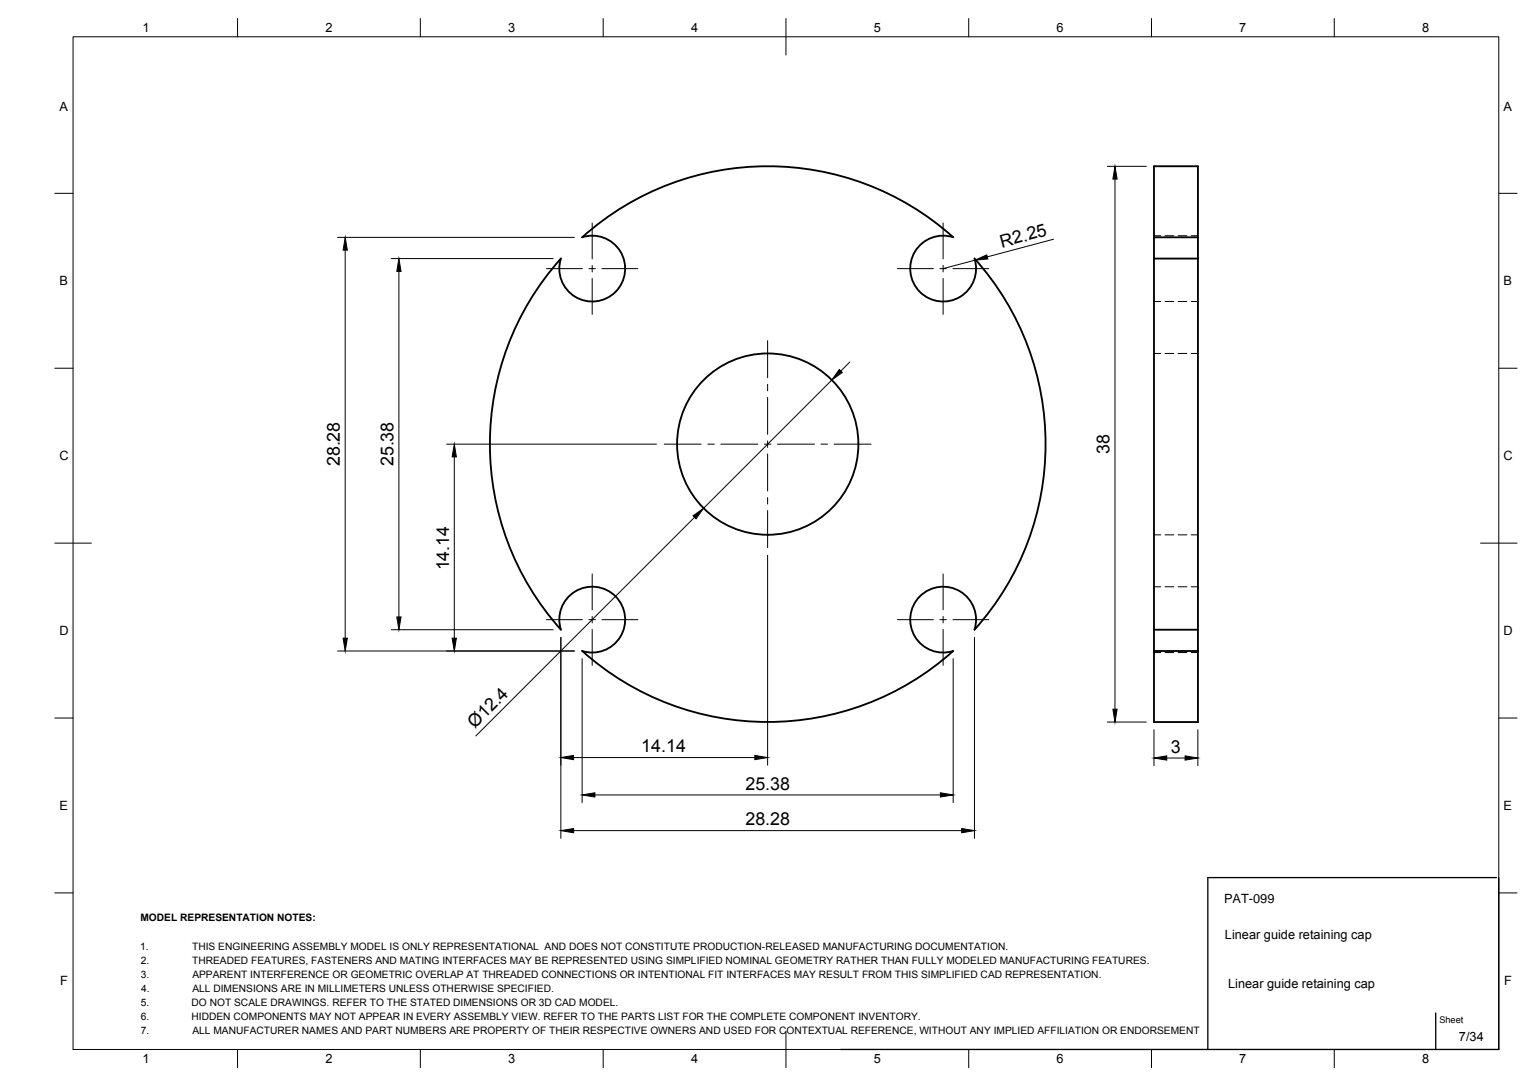
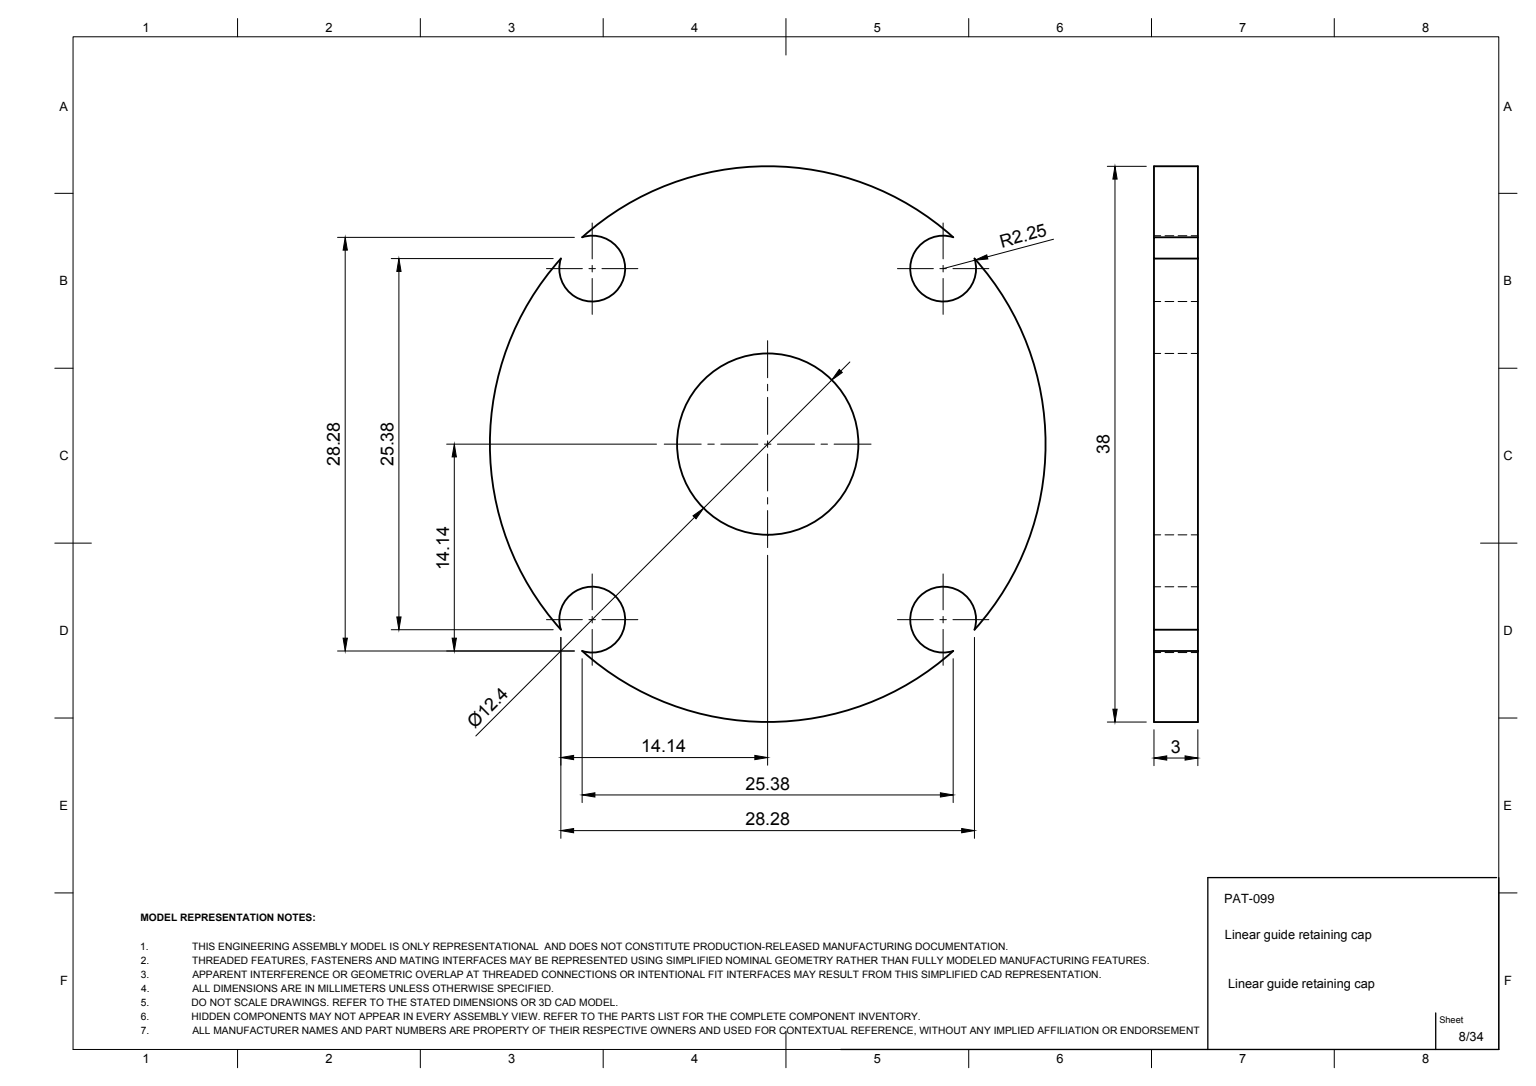
ISO-10303-21;
HEADER;
/* Generated by software containing ST-Developer
 * from STEP Tools, Inc. (www.steptools.com) 
 */

FILE_DESCRIPTION(
/* description */ ('PAT-099'),
/* implementation_level */ '2;1');

FILE_NAME(
/* name */ 'Linear guide retaining cap.step',
/* time_stamp */ '2026-10-29T17:25:42-07:00',
/* author */ (''),
/* organization */ (''),
/* preprocessor_version */ 'ST-DEVELOPER v20.2',
/* originating_system */ 'Autodesk Translation Framework v15.17.0.0',
/* authorisation */ '');

FILE_SCHEMA (('AUTOMOTIVE_DESIGN { 1 0 10303 214 3 1 1 }'));
ENDSEC;

DATA;
#10=MECHANICAL_DESIGN_GEOMETRIC_PRESENTATION_REPRESENTATION('',(#339),#11035);
#289=SHAPE_REPRESENTATION_RELATIONSHIP('SRR','None',#11157,#314);
#314=ADVANCED_BREP_SHAPE_REPRESENTATION('',(#372),#11007);
#339=STYLED_ITEM('',(#11379),#372);
#372=MANIFOLD_SOLID_BREP('Body1',#4707);
#441=FACE_BOUND('',#1018,.T.);
#442=FACE_BOUND('',#1025,.T.);
#537=PLANE('',#5096);
#538=PLANE('',#5112);
#692=FACE_OUTER_BOUND('',#1013,.T.);
#693=FACE_OUTER_BOUND('',#1014,.T.);
#694=FACE_OUTER_BOUND('',#1015,.T.);
#695=FACE_OUTER_BOUND('',#1016,.T.);
#696=FACE_OUTER_BOUND('',#1017,.T.);
#697=FACE_OUTER_BOUND('',#1019,.T.);
#698=FACE_OUTER_BOUND('',#1020,.T.);
#699=FACE_OUTER_BOUND('',#1021,.T.);
#700=FACE_OUTER_BOUND('',#1022,.T.);
#701=FACE_OUTER_BOUND('',#1023,.T.);
#702=FACE_OUTER_BOUND('',#1024,.T.);
#1013=EDGE_LOOP('',(#3313,#3314,#3315,#3316));
#1014=EDGE_LOOP('',(#3317,#3318,#3319,#3320));
#1015=EDGE_LOOP('',(#3321,#3322,#3323,#3324));
#1016=EDGE_LOOP('',(#3325,#3326,#3327,#3328));
#1017=EDGE_LOOP('',(#3329,#3330,#3331,#3332,#3333,#3334,#3335,#3336));
#1018=EDGE_LOOP('',(#3337));
#1019=EDGE_LOOP('',(#3338,#3339,#3340,#3341));
#1020=EDGE_LOOP('',(#3342,#3343,#3344,#3345));
#1021=EDGE_LOOP('',(#3346,#3347,#3348,#3349));
#1022=EDGE_LOOP('',(#3350,#3351,#3352,#3353));
#1023=EDGE_LOOP('',(#3354,#3355,#3356,#3357));
#1024=EDGE_LOOP('',(#3358,#3359,#3360,#3361,#3362,#3363,#3364,#3365));
#1025=EDGE_LOOP('',(#3366));
#1386=LINE('',#7806,#1638);
#1387=LINE('',#7810,#1639);
#1388=LINE('',#7815,#1640);
#1389=LINE('',#7819,#1641);
#1390=LINE('',#7824,#1642);
#1391=LINE('',#7828,#1643);
#1392=LINE('',#7833,#1644);
#1393=LINE('',#7837,#1645);
#1394=LINE('',#7857,#1646);
#1638=VECTOR('',#5849,1.);
#1639=VECTOR('',#5852,1.);
#1640=VECTOR('',#5857,1.);
#1641=VECTOR('',#5860,1.);
#1642=VECTOR('',#5865,1.);
#1643=VECTOR('',#5868,1.);
#1644=VECTOR('',#5873,1.);
#1645=VECTOR('',#5876,1.);
#1646=VECTOR('',#5911,0.62);
#1877=CIRCLE('',#5085,0.225);
#1878=CIRCLE('',#5086,0.225);
#1879=CIRCLE('',#5088,0.225);
#1880=CIRCLE('',#5089,0.225);
#1881=CIRCLE('',#5091,0.225);
#1882=CIRCLE('',#5092,0.225);
#1883=CIRCLE('',#5094,0.225);
#1884=CIRCLE('',#5095,0.225);
#1885=CIRCLE('',#5097,1.9);
#1886=CIRCLE('',#5098,1.9);
#1887=CIRCLE('',#5099,1.9);
#1888=CIRCLE('',#5100,1.9);
#1889=CIRCLE('',#5101,0.62);
#1890=CIRCLE('',#5103,1.9);
#1891=CIRCLE('',#5105,1.9);
#1892=CIRCLE('',#5107,1.9);
#1893=CIRCLE('',#5109,1.9);
#1894=CIRCLE('',#5111,0.62);
#2202=VERTEX_POINT('',#7804);
#2203=VERTEX_POINT('',#7805);
#2204=VERTEX_POINT('',#7807);
#2205=VERTEX_POINT('',#7809);
#2206=VERTEX_POINT('',#7813);
#2207=VERTEX_POINT('',#7814);
#2208=VERTEX_POINT('',#7816);
#2209=VERTEX_POINT('',#7818);
#2210=VERTEX_POINT('',#7822);
#2211=VERTEX_POINT('',#7823);
#2212=VERTEX_POINT('',#7825);
#2213=VERTEX_POINT('',#7827);
#2214=VERTEX_POINT('',#7831);
#2215=VERTEX_POINT('',#7832);
#2216=VERTEX_POINT('',#7834);
#2217=VERTEX_POINT('',#7836);
#2218=VERTEX_POINT('',#7844);
#2219=VERTEX_POINT('',#7855);
#2633=EDGE_CURVE('',#2202,#2203,#1386,.T.);
#2634=EDGE_CURVE('',#2204,#2202,#1877,.T.);
#2635=EDGE_CURVE('',#2205,#2204,#1387,.T.);
#2636=EDGE_CURVE('',#2203,#2205,#1878,.T.);
#2637=EDGE_CURVE('',#2206,#2207,#1388,.T.);
#2638=EDGE_CURVE('',#2208,#2206,#1879,.T.);
#2639=EDGE_CURVE('',#2209,#2208,#1389,.T.);
#2640=EDGE_CURVE('',#2207,#2209,#1880,.T.);
#2641=EDGE_CURVE('',#2210,#2211,#1390,.T.);
#2642=EDGE_CURVE('',#2212,#2210,#1881,.T.);
#2643=EDGE_CURVE('',#2213,#2212,#1391,.T.);
#2644=EDGE_CURVE('',#2211,#2213,#1882,.T.);
#2645=EDGE_CURVE('',#2214,#2215,#1392,.T.);
#2646=EDGE_CURVE('',#2216,#2214,#1883,.T.);
#2647=EDGE_CURVE('',#2217,#2216,#1393,.T.);
#2648=EDGE_CURVE('',#2215,#2217,#1884,.T.);
#2649=EDGE_CURVE('',#2212,#2202,#1885,.T.);
#2650=EDGE_CURVE('',#2208,#2210,#1886,.T.);
#2651=EDGE_CURVE('',#2216,#2206,#1887,.T.);
#2652=EDGE_CURVE('',#2204,#2214,#1888,.T.);
#2653=EDGE_CURVE('',#2218,#2218,#1889,.T.);
#2654=EDGE_CURVE('',#2217,#2207,#1890,.T.);
#2655=EDGE_CURVE('',#2209,#2211,#1891,.T.);
#2656=EDGE_CURVE('',#2213,#2203,#1892,.T.);
#2657=EDGE_CURVE('',#2205,#2215,#1893,.T.);
#2658=EDGE_CURVE('',#2219,#2219,#1894,.T.);
#2659=EDGE_CURVE('',#2219,#2218,#1394,.T.);
#3313=ORIENTED_EDGE('',*,*,#2633,.F.);
#3314=ORIENTED_EDGE('',*,*,#2634,.F.);
#3315=ORIENTED_EDGE('',*,*,#2635,.F.);
#3316=ORIENTED_EDGE('',*,*,#2636,.F.);
#3317=ORIENTED_EDGE('',*,*,#2637,.F.);
#3318=ORIENTED_EDGE('',*,*,#2638,.F.);
#3319=ORIENTED_EDGE('',*,*,#2639,.F.);
#3320=ORIENTED_EDGE('',*,*,#2640,.F.);
#3321=ORIENTED_EDGE('',*,*,#2641,.F.);
#3322=ORIENTED_EDGE('',*,*,#2642,.F.);
#3323=ORIENTED_EDGE('',*,*,#2643,.F.);
#3324=ORIENTED_EDGE('',*,*,#2644,.F.);
#3325=ORIENTED_EDGE('',*,*,#2645,.F.);
#3326=ORIENTED_EDGE('',*,*,#2646,.F.);
#3327=ORIENTED_EDGE('',*,*,#2647,.F.);
#3328=ORIENTED_EDGE('',*,*,#2648,.F.);
#3329=ORIENTED_EDGE('',*,*,#2634,.T.);
#3330=ORIENTED_EDGE('',*,*,#2649,.F.);
#3331=ORIENTED_EDGE('',*,*,#2642,.T.);
#3332=ORIENTED_EDGE('',*,*,#2650,.F.);
#3333=ORIENTED_EDGE('',*,*,#2638,.T.);
#3334=ORIENTED_EDGE('',*,*,#2651,.F.);
#3335=ORIENTED_EDGE('',*,*,#2646,.T.);
#3336=ORIENTED_EDGE('',*,*,#2652,.F.);
#3337=ORIENTED_EDGE('',*,*,#2653,.F.);
#3338=ORIENTED_EDGE('',*,*,#2637,.T.);
#3339=ORIENTED_EDGE('',*,*,#2654,.F.);
#3340=ORIENTED_EDGE('',*,*,#2647,.T.);
#3341=ORIENTED_EDGE('',*,*,#2651,.T.);
#3342=ORIENTED_EDGE('',*,*,#2639,.T.);
#3343=ORIENTED_EDGE('',*,*,#2650,.T.);
#3344=ORIENTED_EDGE('',*,*,#2641,.T.);
#3345=ORIENTED_EDGE('',*,*,#2655,.F.);
#3346=ORIENTED_EDGE('',*,*,#2633,.T.);
#3347=ORIENTED_EDGE('',*,*,#2656,.F.);
#3348=ORIENTED_EDGE('',*,*,#2643,.T.);
#3349=ORIENTED_EDGE('',*,*,#2649,.T.);
#3350=ORIENTED_EDGE('',*,*,#2635,.T.);
#3351=ORIENTED_EDGE('',*,*,#2652,.T.);
#3352=ORIENTED_EDGE('',*,*,#2645,.T.);
#3353=ORIENTED_EDGE('',*,*,#2657,.F.);
#3354=ORIENTED_EDGE('',*,*,#2658,.F.);
#3355=ORIENTED_EDGE('',*,*,#2659,.T.);
#3356=ORIENTED_EDGE('',*,*,#2653,.T.);
#3357=ORIENTED_EDGE('',*,*,#2659,.F.);
#3358=ORIENTED_EDGE('',*,*,#2636,.T.);
#3359=ORIENTED_EDGE('',*,*,#2657,.T.);
#3360=ORIENTED_EDGE('',*,*,#2648,.T.);
#3361=ORIENTED_EDGE('',*,*,#2654,.T.);
#3362=ORIENTED_EDGE('',*,*,#2640,.T.);
#3363=ORIENTED_EDGE('',*,*,#2655,.T.);
#3364=ORIENTED_EDGE('',*,*,#2644,.T.);
#3365=ORIENTED_EDGE('',*,*,#2656,.T.);
#3366=ORIENTED_EDGE('',*,*,#2658,.T.);
#4328=CYLINDRICAL_SURFACE('',#5084,0.225);
#4329=CYLINDRICAL_SURFACE('',#5087,0.225);
#4330=CYLINDRICAL_SURFACE('',#5090,0.225);
#4331=CYLINDRICAL_SURFACE('',#5093,0.225);
#4332=CYLINDRICAL_SURFACE('',#5102,1.9);
#4333=CYLINDRICAL_SURFACE('',#5104,1.9);
#4334=CYLINDRICAL_SURFACE('',#5106,1.9);
#4335=CYLINDRICAL_SURFACE('',#5108,1.9);
#4336=CYLINDRICAL_SURFACE('',#5110,0.62);
#4457=ADVANCED_FACE('',(#692),#4328,.F.);
#4458=ADVANCED_FACE('',(#693),#4329,.F.);
#4459=ADVANCED_FACE('',(#694),#4330,.F.);
#4460=ADVANCED_FACE('',(#695),#4331,.F.);
#4461=ADVANCED_FACE('',(#696,#441),#537,.F.);
#4462=ADVANCED_FACE('',(#697),#4332,.T.);
#4463=ADVANCED_FACE('',(#698),#4333,.T.);
#4464=ADVANCED_FACE('',(#699),#4334,.T.);
#4465=ADVANCED_FACE('',(#700),#4335,.T.);
#4466=ADVANCED_FACE('',(#701),#4336,.F.);
#4467=ADVANCED_FACE('',(#702,#442),#538,.T.);
#4707=CLOSED_SHELL('',(#4457,#4458,#4459,#4460,#4461,#4462,#4463,#4464,
#4465,#4466,#4467));
#5083=AXIS2_PLACEMENT_3D('',#7802,#5845,#5846);
#5084=AXIS2_PLACEMENT_3D('',#7803,#5847,#5848);
#5085=AXIS2_PLACEMENT_3D('',#7808,#5850,#5851);
#5086=AXIS2_PLACEMENT_3D('',#7811,#5853,#5854);
#5087=AXIS2_PLACEMENT_3D('',#7812,#5855,#5856);
#5088=AXIS2_PLACEMENT_3D('',#7817,#5858,#5859);
#5089=AXIS2_PLACEMENT_3D('',#7820,#5861,#5862);
#5090=AXIS2_PLACEMENT_3D('',#7821,#5863,#5864);
#5091=AXIS2_PLACEMENT_3D('',#7826,#5866,#5867);
#5092=AXIS2_PLACEMENT_3D('',#7829,#5869,#5870);
#5093=AXIS2_PLACEMENT_3D('',#7830,#5871,#5872);
#5094=AXIS2_PLACEMENT_3D('',#7835,#5874,#5875);
#5095=AXIS2_PLACEMENT_3D('',#7838,#5877,#5878);
#5096=AXIS2_PLACEMENT_3D('',#7839,#5879,#5880);
#5097=AXIS2_PLACEMENT_3D('',#7840,#5881,#5882);
#5098=AXIS2_PLACEMENT_3D('',#7841,#5883,#5884);
#5099=AXIS2_PLACEMENT_3D('',#7842,#5885,#5886);
#5100=AXIS2_PLACEMENT_3D('',#7843,#5887,#5888);
#5101=AXIS2_PLACEMENT_3D('',#7845,#5889,#5890);
#5102=AXIS2_PLACEMENT_3D('',#7846,#5891,#5892);
#5103=AXIS2_PLACEMENT_3D('',#7847,#5893,#5894);
#5104=AXIS2_PLACEMENT_3D('',#7848,#5895,#5896);
#5105=AXIS2_PLACEMENT_3D('',#7849,#5897,#5898);
#5106=AXIS2_PLACEMENT_3D('',#7850,#5899,#5900);
#5107=AXIS2_PLACEMENT_3D('',#7851,#5901,#5902);
#5108=AXIS2_PLACEMENT_3D('',#7852,#5903,#5904);
#5109=AXIS2_PLACEMENT_3D('',#7853,#5905,#5906);
#5110=AXIS2_PLACEMENT_3D('',#7854,#5907,#5908);
#5111=AXIS2_PLACEMENT_3D('',#7856,#5909,#5910);
#5112=AXIS2_PLACEMENT_3D('',#7858,#5912,#5913);
#5845=DIRECTION('axis',(0.,0.,1.));
#5846=DIRECTION('refdir',(1.,0.,0.));
#5847=DIRECTION('center_axis',(1.,0.,0.));
#5848=DIRECTION('ref_axis',(0.,-0.707106781186549,0.707106781186546));
#5849=DIRECTION('',(1.,0.,0.));
#5850=DIRECTION('center_axis',(1.,0.,0.));
#5851=DIRECTION('ref_axis',(0.,0.,-1.));
#5852=DIRECTION('',(-1.,0.,0.));
#5853=DIRECTION('center_axis',(-1.,0.,0.));
#5854=DIRECTION('ref_axis',(0.,0.,-1.));
#5855=DIRECTION('center_axis',(1.,0.,0.));
#5856=DIRECTION('ref_axis',(0.,0.707106781186548,-0.707106781186547));
#5857=DIRECTION('',(1.,0.,0.));
#5858=DIRECTION('center_axis',(1.,0.,0.));
#5859=DIRECTION('ref_axis',(0.,0.,-1.));
#5860=DIRECTION('',(-1.,0.,0.));
#5861=DIRECTION('center_axis',(-1.,0.,0.));
#5862=DIRECTION('ref_axis',(0.,0.,-1.));
#5863=DIRECTION('center_axis',(1.,0.,0.));
#5864=DIRECTION('ref_axis',(0.,0.707106781186549,0.707106781186546));
#5865=DIRECTION('',(1.,0.,0.));
#5866=DIRECTION('center_axis',(1.,0.,0.));
#5867=DIRECTION('ref_axis',(0.,0.,-1.));
#5868=DIRECTION('',(-1.,0.,0.));
#5869=DIRECTION('center_axis',(-1.,0.,0.));
#5870=DIRECTION('ref_axis',(0.,0.,-1.));
#5871=DIRECTION('center_axis',(1.,0.,0.));
#5872=DIRECTION('ref_axis',(0.,-0.707106781186547,-0.707106781186548));
#5873=DIRECTION('',(1.,0.,0.));
#5874=DIRECTION('center_axis',(1.,0.,0.));
#5875=DIRECTION('ref_axis',(0.,0.,-1.));
#5876=DIRECTION('',(-1.,0.,0.));
#5877=DIRECTION('center_axis',(-1.,0.,0.));
#5878=DIRECTION('ref_axis',(0.,0.,-1.));
#5879=DIRECTION('center_axis',(1.,0.,0.));
#5880=DIRECTION('ref_axis',(0.,0.,-1.));
#5881=DIRECTION('center_axis',(1.,0.,0.));
#5882=DIRECTION('ref_axis',(0.,0.,-1.));
#5883=DIRECTION('center_axis',(1.,0.,0.));
#5884=DIRECTION('ref_axis',(0.,0.,-1.));
#5885=DIRECTION('center_axis',(1.,0.,0.));
#5886=DIRECTION('ref_axis',(0.,0.,-1.));
#5887=DIRECTION('center_axis',(1.,0.,0.));
#5888=DIRECTION('ref_axis',(0.,0.,-1.));
#5889=DIRECTION('center_axis',(-1.,0.,0.));
#5890=DIRECTION('ref_axis',(0.,0.,-1.));
#5891=DIRECTION('center_axis',(1.,0.,0.));
#5892=DIRECTION('ref_axis',(0.,-1.22464679914735E-16,1.));
#5893=DIRECTION('center_axis',(1.,0.,0.));
#5894=DIRECTION('ref_axis',(0.,0.,-1.));
#5895=DIRECTION('center_axis',(1.,0.,0.));
#5896=DIRECTION('ref_axis',(0.,0.,-1.));
#5897=DIRECTION('center_axis',(1.,0.,0.));
#5898=DIRECTION('ref_axis',(0.,0.,-1.));
#5899=DIRECTION('center_axis',(1.,0.,0.));
#5900=DIRECTION('ref_axis',(0.,0.,-1.));
#5901=DIRECTION('center_axis',(1.,0.,0.));
#5902=DIRECTION('ref_axis',(0.,0.,-1.));
#5903=DIRECTION('center_axis',(1.,0.,0.));
#5904=DIRECTION('ref_axis',(0.,0.,-1.));
#5905=DIRECTION('center_axis',(1.,0.,0.));
#5906=DIRECTION('ref_axis',(0.,0.,-1.));
#5907=DIRECTION('center_axis',(1.,0.,0.));
#5908=DIRECTION('ref_axis',(0.,0.,-1.));
#5909=DIRECTION('center_axis',(-1.,0.,0.));
#5910=DIRECTION('ref_axis',(0.,0.,-1.));
#5911=DIRECTION('',(-1.,0.,0.));
#5912=DIRECTION('center_axis',(1.,0.,0.));
#5913=DIRECTION('ref_axis',(0.,0.,-1.));
#7802=CARTESIAN_POINT('',(0.,0.,0.));
#7803=CARTESIAN_POINT('Origin',(9.6,1.2,4.05));
#7804=CARTESIAN_POINT('',(9.7,1.26887332488551,3.83580040821884));
#7805=CARTESIAN_POINT('',(10.,1.26887332488551,3.83580040821884));
#7806=CARTESIAN_POINT('',(9.6,1.26887332488551,3.83580040821884));
#7807=CARTESIAN_POINT('',(9.7,1.41419959178116,3.98112667511449));
#7808=CARTESIAN_POINT('Origin',(9.7,1.2,4.05));
#7809=CARTESIAN_POINT('',(10.,1.41419959178116,3.98112667511449));
#7810=CARTESIAN_POINT('',(9.6,1.41419959178116,3.98112667511449));
#7811=CARTESIAN_POINT('Origin',(10.,1.2,4.05));
#7812=CARTESIAN_POINT('Origin',(9.6,-1.2,6.45));
#7813=CARTESIAN_POINT('',(9.7,-1.26887332488551,6.66419959178116));
#7814=CARTESIAN_POINT('',(10.,-1.26887332488551,6.66419959178116));
#7815=CARTESIAN_POINT('',(9.6,-1.26887332488551,6.66419959178116));
#7816=CARTESIAN_POINT('',(9.7,-1.41419959178116,6.51887332488551));
#7817=CARTESIAN_POINT('Origin',(9.7,-1.2,6.45));
#7818=CARTESIAN_POINT('',(10.,-1.41419959178116,6.51887332488551));
#7819=CARTESIAN_POINT('',(9.6,-1.41419959178116,6.51887332488551));
#7820=CARTESIAN_POINT('Origin',(10.,-1.2,6.45));
#7821=CARTESIAN_POINT('Origin',(9.6,-1.2,4.05));
#7822=CARTESIAN_POINT('',(9.7,-1.41419959178116,3.98112667511449));
#7823=CARTESIAN_POINT('',(10.,-1.41419959178116,3.98112667511449));
#7824=CARTESIAN_POINT('',(9.6,-1.41419959178116,3.98112667511449));
#7825=CARTESIAN_POINT('',(9.7,-1.26887332488551,3.83580040821884));
#7826=CARTESIAN_POINT('Origin',(9.7,-1.2,4.05));
#7827=CARTESIAN_POINT('',(10.,-1.26887332488551,3.83580040821884));
#7828=CARTESIAN_POINT('',(9.6,-1.26887332488551,3.83580040821884));
#7829=CARTESIAN_POINT('Origin',(10.,-1.2,4.05));
#7830=CARTESIAN_POINT('Origin',(9.6,1.2,6.45));
#7831=CARTESIAN_POINT('',(9.7,1.41419959178116,6.51887332488551));
#7832=CARTESIAN_POINT('',(10.,1.41419959178116,6.51887332488551));
#7833=CARTESIAN_POINT('',(9.6,1.41419959178116,6.51887332488551));
#7834=CARTESIAN_POINT('',(9.7,1.26887332488551,6.66419959178116));
#7835=CARTESIAN_POINT('Origin',(9.7,1.2,6.45));
#7836=CARTESIAN_POINT('',(10.,1.26887332488551,6.66419959178116));
#7837=CARTESIAN_POINT('',(9.6,1.26887332488551,6.66419959178116));
#7838=CARTESIAN_POINT('Origin',(10.,1.2,6.45));
#7839=CARTESIAN_POINT('Origin',(9.7,0.,5.25));
#7840=CARTESIAN_POINT('Origin',(9.7,0.,5.25));
#7841=CARTESIAN_POINT('Origin',(9.7,0.,5.25));
#7842=CARTESIAN_POINT('Origin',(9.7,0.,5.25));
#7843=CARTESIAN_POINT('Origin',(9.7,0.,5.25));
#7844=CARTESIAN_POINT('',(9.7,-7.59281015471359E-17,5.87));
#7845=CARTESIAN_POINT('Origin',(9.7,0.,5.25));
#7846=CARTESIAN_POINT('Origin',(9.7,0.,5.25));
#7847=CARTESIAN_POINT('Origin',(10.,0.,5.25));
#7848=CARTESIAN_POINT('Origin',(9.7,0.,5.25));
#7849=CARTESIAN_POINT('Origin',(10.,0.,5.25));
#7850=CARTESIAN_POINT('Origin',(9.7,0.,5.25));
#7851=CARTESIAN_POINT('Origin',(10.,0.,5.25));
#7852=CARTESIAN_POINT('Origin',(9.7,0.,5.25));
#7853=CARTESIAN_POINT('Origin',(10.,0.,5.25));
#7854=CARTESIAN_POINT('Origin',(9.7,0.,5.25));
#7855=CARTESIAN_POINT('',(10.,-7.59281015471359E-17,5.87));
#7856=CARTESIAN_POINT('Origin',(10.,0.,5.25));
#7857=CARTESIAN_POINT('',(9.7,-7.59281015471359E-17,5.87));
#7858=CARTESIAN_POINT('Origin',(10.,0.,5.25));
#10974=UNCERTAINTY_MEASURE_WITH_UNIT(LENGTH_MEASURE(0.001),#11036,
'DISTANCE_ACCURACY_VALUE',
'Maximum model space distance between geometric entities at asserted c
onnectivities');
#11002=UNCERTAINTY_MEASURE_WITH_UNIT(LENGTH_MEASURE(0.001),#11036,
'DISTANCE_ACCURACY_VALUE',
'Maximum model space distance between geometric entities at asserted c
onnectivities');
#11007=(
GEOMETRIC_REPRESENTATION_CONTEXT(3)
GLOBAL_UNCERTAINTY_ASSIGNED_CONTEXT((#10974))
GLOBAL_UNIT_ASSIGNED_CONTEXT((#11036,#11038,#11039))
REPRESENTATION_CONTEXT('','3D')
);
#11035=(
GEOMETRIC_REPRESENTATION_CONTEXT(3)
GLOBAL_UNCERTAINTY_ASSIGNED_CONTEXT((#11002))
GLOBAL_UNIT_ASSIGNED_CONTEXT((#11036,#11038,#11039))
REPRESENTATION_CONTEXT('','3D')
);
#11036=(
LENGTH_UNIT()
NAMED_UNIT(*)
SI_UNIT(.CENTI.,.METRE.)
);
#11038=(
NAMED_UNIT(*)
PLANE_ANGLE_UNIT()
SI_UNIT($,.RADIAN.)
);
#11039=(
NAMED_UNIT(*)
SI_UNIT($,.STERADIAN.)
SOLID_ANGLE_UNIT()
);
#11044=SHAPE_DEFINITION_REPRESENTATION(#11076,#11157);
#11076=PRODUCT_DEFINITION_SHAPE('',$,#11190);
#11157=SHAPE_REPRESENTATION('',(#5083),#11007);
#11185=PRODUCT_DEFINITION_CONTEXT('part definition',#11283,'design');
#11190=PRODUCT_DEFINITION('Linear guide retaining cap',
'Linear guide retaining cap',#11222,#11185);
#11222=PRODUCT_DEFINITION_FORMATION('',$,#11289);
#11283=APPLICATION_CONTEXT(
'Core Data for Automotive Mechanical Design Process');
#11284=PRODUCT_CONTEXT('part definition',#11283,'mechanical');
#11289=PRODUCT('Linear guide retaining cap',
'Linear guide retaining cap','Linear guide retaining cap',(#11284));
#11373=COLOUR_RGB('Sky Blue',0.24,0.69,0.87);
#11374=FILL_AREA_STYLE_COLOUR('',#11373);
#11375=FILL_AREA_STYLE('',(#11374));
#11376=SURFACE_STYLE_FILL_AREA(#11375);
#11377=SURFACE_SIDE_STYLE('',(#11376));
#11378=SURFACE_STYLE_USAGE(.BOTH.,#11377);
#11379=PRESENTATION_STYLE_ASSIGNMENT((#11378));
ENDSEC;
END-ISO-10303-21;
